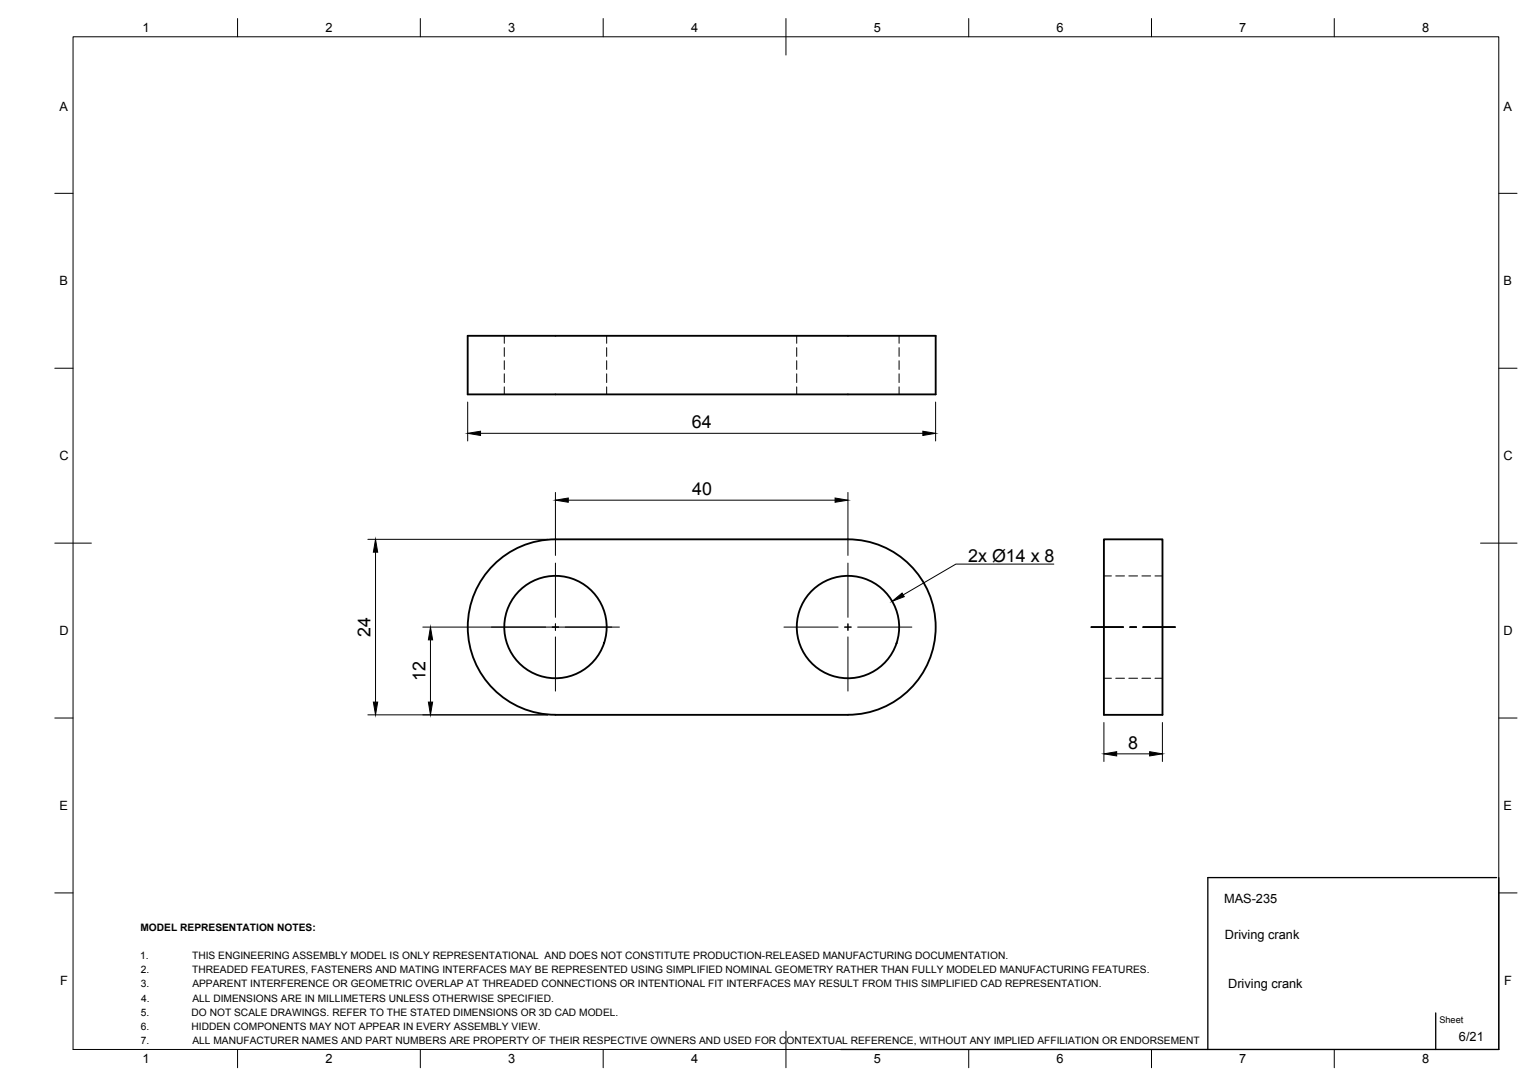
ISO-10303-21;
HEADER;
/* Generated by software containing ST-Developer
 * from STEP Tools, Inc. (www.steptools.com) 
 */

FILE_DESCRIPTION(
/* description */ ('Independent Whitworth quick-return mechanism. Crank radius40, ground-
center spacing80, lever180, connecting rod160, output guide X200. Nomi
nal stroke180 and long/short phase ratio2. Retained guide rods, replac
eable bearing sleeves and captured sliding shoe. No load or production
 rating assigned.'),
/* implementation_level */ '2;1');

FILE_NAME(
/* name */ 'Driving crank.step',
/* time_stamp */ '2026-11-09T18:22:56-08:00',
/* author */ (''),
/* organization */ (''),
/* preprocessor_version */ 'ST-DEVELOPER v20.2',
/* originating_system */ 'Autodesk Translation Framework v15.17.0.0',
/* authorisation */ '');

FILE_SCHEMA (('AUTOMOTIVE_DESIGN { 1 0 10303 214 3 1 1 }'));
ENDSEC;

DATA;
#10=MECHANICAL_DESIGN_GEOMETRIC_PRESENTATION_REPRESENTATION('',(#222),#4388);
#182=SHAPE_REPRESENTATION_RELATIONSHIP('SRR','None',#4481,#202);
#202=ADVANCED_BREP_SHAPE_REPRESENTATION('',(#242),#4371);
#222=STYLED_ITEM('',(#4589),#242);
#242=MANIFOLD_SOLID_BREP('Body1',#2327);
#267=FACE_BOUND('',#583,.T.);
#268=FACE_BOUND('',#584,.T.);
#269=FACE_BOUND('',#586,.T.);
#270=FACE_BOUND('',#587,.T.);
#329=PLANE('',#2604);
#330=PLANE('',#2608);
#331=PLANE('',#2612);
#332=PLANE('',#2613);
#421=FACE_OUTER_BOUND('',#576,.T.);
#422=FACE_OUTER_BOUND('',#577,.T.);
#423=FACE_OUTER_BOUND('',#578,.T.);
#424=FACE_OUTER_BOUND('',#579,.T.);
#425=FACE_OUTER_BOUND('',#580,.T.);
#426=FACE_OUTER_BOUND('',#581,.T.);
#427=FACE_OUTER_BOUND('',#582,.T.);
#428=FACE_OUTER_BOUND('',#585,.T.);
#576=EDGE_LOOP('',(#1654,#1655,#1656,#1657));
#577=EDGE_LOOP('',(#1658,#1659,#1660,#1661));
#578=EDGE_LOOP('',(#1662,#1663,#1664,#1665));
#579=EDGE_LOOP('',(#1666,#1667,#1668,#1669));
#580=EDGE_LOOP('',(#1670,#1671,#1672,#1673));
#581=EDGE_LOOP('',(#1674,#1675,#1676,#1677));
#582=EDGE_LOOP('',(#1678,#1679,#1680,#1681));
#583=EDGE_LOOP('',(#1682));
#584=EDGE_LOOP('',(#1683));
#585=EDGE_LOOP('',(#1684,#1685,#1686,#1687));
#586=EDGE_LOOP('',(#1688));
#587=EDGE_LOOP('',(#1689));
#777=LINE('',#3775,#916);
#778=LINE('',#3781,#917);
#779=LINE('',#3786,#918);
#780=LINE('',#3788,#919);
#781=LINE('',#3790,#920);
#782=LINE('',#3791,#921);
#783=LINE('',#3797,#922);
#784=LINE('',#3800,#923);
#785=LINE('',#3802,#924);
#786=LINE('',#3803,#925);
#916=VECTOR('',#2985,7.);
#917=VECTOR('',#2992,7.);
#918=VECTOR('',#2997,10.);
#919=VECTOR('',#2998,10.);
#920=VECTOR('',#2999,10.);
#921=VECTOR('',#3000,10.);
#922=VECTOR('',#3007,10.);
#923=VECTOR('',#3010,10.);
#924=VECTOR('',#3011,10.);
#925=VECTOR('',#3012,10.);
#1049=CIRCLE('',#2599,7.);
#1050=CIRCLE('',#2600,7.);
#1051=CIRCLE('',#2602,7.);
#1052=CIRCLE('',#2603,7.);
#1053=CIRCLE('',#2606,12.);
#1054=CIRCLE('',#2607,12.);
#1055=CIRCLE('',#2610,12.);
#1056=CIRCLE('',#2611,12.);
#1179=VERTEX_POINT('',#3772);
#1180=VERTEX_POINT('',#3774);
#1181=VERTEX_POINT('',#3778);
#1182=VERTEX_POINT('',#3780);
#1183=VERTEX_POINT('',#3784);
#1184=VERTEX_POINT('',#3785);
#1185=VERTEX_POINT('',#3787);
#1186=VERTEX_POINT('',#3789);
#1187=VERTEX_POINT('',#3793);
#1188=VERTEX_POINT('',#3795);
#1189=VERTEX_POINT('',#3799);
#1190=VERTEX_POINT('',#3801);
#1363=EDGE_CURVE('',#1179,#1179,#1049,.T.);
#1364=EDGE_CURVE('',#1179,#1180,#777,.T.);
#1365=EDGE_CURVE('',#1180,#1180,#1050,.T.);
#1366=EDGE_CURVE('',#1181,#1181,#1051,.T.);
#1367=EDGE_CURVE('',#1181,#1182,#778,.T.);
#1368=EDGE_CURVE('',#1182,#1182,#1052,.T.);
#1369=EDGE_CURVE('',#1183,#1184,#779,.T.);
#1370=EDGE_CURVE('',#1184,#1185,#780,.T.);
#1371=EDGE_CURVE('',#1186,#1185,#781,.T.);
#1372=EDGE_CURVE('',#1183,#1186,#782,.T.);
#1373=EDGE_CURVE('',#1187,#1183,#1053,.T.);
#1374=EDGE_CURVE('',#1188,#1186,#1054,.T.);
#1375=EDGE_CURVE('',#1187,#1188,#783,.T.);
#1376=EDGE_CURVE('',#1189,#1187,#784,.T.);
#1377=EDGE_CURVE('',#1190,#1188,#785,.T.);
#1378=EDGE_CURVE('',#1189,#1190,#786,.T.);
#1379=EDGE_CURVE('',#1184,#1189,#1055,.T.);
#1380=EDGE_CURVE('',#1185,#1190,#1056,.T.);
#1654=ORIENTED_EDGE('',*,*,#1363,.F.);
#1655=ORIENTED_EDGE('',*,*,#1364,.T.);
#1656=ORIENTED_EDGE('',*,*,#1365,.F.);
#1657=ORIENTED_EDGE('',*,*,#1364,.F.);
#1658=ORIENTED_EDGE('',*,*,#1366,.F.);
#1659=ORIENTED_EDGE('',*,*,#1367,.T.);
#1660=ORIENTED_EDGE('',*,*,#1368,.F.);
#1661=ORIENTED_EDGE('',*,*,#1367,.F.);
#1662=ORIENTED_EDGE('',*,*,#1369,.T.);
#1663=ORIENTED_EDGE('',*,*,#1370,.T.);
#1664=ORIENTED_EDGE('',*,*,#1371,.F.);
#1665=ORIENTED_EDGE('',*,*,#1372,.F.);
#1666=ORIENTED_EDGE('',*,*,#1373,.T.);
#1667=ORIENTED_EDGE('',*,*,#1372,.T.);
#1668=ORIENTED_EDGE('',*,*,#1374,.F.);
#1669=ORIENTED_EDGE('',*,*,#1375,.F.);
#1670=ORIENTED_EDGE('',*,*,#1376,.T.);
#1671=ORIENTED_EDGE('',*,*,#1375,.T.);
#1672=ORIENTED_EDGE('',*,*,#1377,.F.);
#1673=ORIENTED_EDGE('',*,*,#1378,.F.);
#1674=ORIENTED_EDGE('',*,*,#1379,.T.);
#1675=ORIENTED_EDGE('',*,*,#1378,.T.);
#1676=ORIENTED_EDGE('',*,*,#1380,.F.);
#1677=ORIENTED_EDGE('',*,*,#1370,.F.);
#1678=ORIENTED_EDGE('',*,*,#1380,.T.);
#1679=ORIENTED_EDGE('',*,*,#1377,.T.);
#1680=ORIENTED_EDGE('',*,*,#1374,.T.);
#1681=ORIENTED_EDGE('',*,*,#1371,.T.);
#1682=ORIENTED_EDGE('',*,*,#1363,.T.);
#1683=ORIENTED_EDGE('',*,*,#1366,.T.);
#1684=ORIENTED_EDGE('',*,*,#1379,.F.);
#1685=ORIENTED_EDGE('',*,*,#1369,.F.);
#1686=ORIENTED_EDGE('',*,*,#1373,.F.);
#1687=ORIENTED_EDGE('',*,*,#1376,.F.);
#1688=ORIENTED_EDGE('',*,*,#1365,.T.);
#1689=ORIENTED_EDGE('',*,*,#1368,.T.);
#2122=CYLINDRICAL_SURFACE('',#2598,7.);
#2123=CYLINDRICAL_SURFACE('',#2601,7.);
#2124=CYLINDRICAL_SURFACE('',#2605,12.);
#2125=CYLINDRICAL_SURFACE('',#2609,12.);
#2193=ADVANCED_FACE('',(#421),#2122,.F.);
#2194=ADVANCED_FACE('',(#422),#2123,.F.);
#2195=ADVANCED_FACE('',(#423),#329,.T.);
#2196=ADVANCED_FACE('',(#424),#2124,.T.);
#2197=ADVANCED_FACE('',(#425),#330,.T.);
#2198=ADVANCED_FACE('',(#426),#2125,.T.);
#2199=ADVANCED_FACE('',(#427,#267,#268),#331,.T.);
#2200=ADVANCED_FACE('',(#428,#269,#270),#332,.F.);
#2327=CLOSED_SHELL('',(#2193,#2194,#2195,#2196,#2197,#2198,#2199,#2200));
#2597=AXIS2_PLACEMENT_3D('',#3770,#2979,#2980);
#2598=AXIS2_PLACEMENT_3D('',#3771,#2981,#2982);
#2599=AXIS2_PLACEMENT_3D('',#3773,#2983,#2984);
#2600=AXIS2_PLACEMENT_3D('',#3776,#2986,#2987);
#2601=AXIS2_PLACEMENT_3D('',#3777,#2988,#2989);
#2602=AXIS2_PLACEMENT_3D('',#3779,#2990,#2991);
#2603=AXIS2_PLACEMENT_3D('',#3782,#2993,#2994);
#2604=AXIS2_PLACEMENT_3D('',#3783,#2995,#2996);
#2605=AXIS2_PLACEMENT_3D('',#3792,#3001,#3002);
#2606=AXIS2_PLACEMENT_3D('',#3794,#3003,#3004);
#2607=AXIS2_PLACEMENT_3D('',#3796,#3005,#3006);
#2608=AXIS2_PLACEMENT_3D('',#3798,#3008,#3009);
#2609=AXIS2_PLACEMENT_3D('',#3804,#3013,#3014);
#2610=AXIS2_PLACEMENT_3D('',#3805,#3015,#3016);
#2611=AXIS2_PLACEMENT_3D('',#3806,#3017,#3018);
#2612=AXIS2_PLACEMENT_3D('',#3807,#3019,#3020);
#2613=AXIS2_PLACEMENT_3D('',#3808,#3021,#3022);
#2979=DIRECTION('axis',(0.,0.,1.));
#2980=DIRECTION('refdir',(1.,0.,0.));
#2981=DIRECTION('center_axis',(0.,0.,-1.));
#2982=DIRECTION('ref_axis',(1.,0.,0.));
#2983=DIRECTION('center_axis',(0.,0.,-1.));
#2984=DIRECTION('ref_axis',(1.,0.,0.));
#2985=DIRECTION('',(0.,0.,-1.));
#2986=DIRECTION('center_axis',(0.,0.,1.));
#2987=DIRECTION('ref_axis',(1.,0.,0.));
#2988=DIRECTION('center_axis',(0.,0.,-1.));
#2989=DIRECTION('ref_axis',(1.,0.,0.));
#2990=DIRECTION('center_axis',(0.,0.,-1.));
#2991=DIRECTION('ref_axis',(1.,0.,0.));
#2992=DIRECTION('',(0.,0.,-1.));
#2993=DIRECTION('center_axis',(0.,0.,1.));
#2994=DIRECTION('ref_axis',(1.,0.,0.));
#2995=DIRECTION('center_axis',(0.,1.,0.));
#2996=DIRECTION('ref_axis',(-1.,0.,0.));
#2997=DIRECTION('',(-1.,0.,0.));
#2998=DIRECTION('',(0.,0.,1.));
#2999=DIRECTION('',(-1.,0.,0.));
#3000=DIRECTION('',(0.,0.,1.));
#3001=DIRECTION('center_axis',(0.,0.,1.));
#3002=DIRECTION('ref_axis',(0.,-1.,0.));
#3003=DIRECTION('center_axis',(0.,0.,1.));
#3004=DIRECTION('ref_axis',(0.,-1.,0.));
#3005=DIRECTION('center_axis',(0.,0.,1.));
#3006=DIRECTION('ref_axis',(0.,-1.,0.));
#3007=DIRECTION('',(0.,0.,1.));
#3008=DIRECTION('center_axis',(0.,-1.,0.));
#3009=DIRECTION('ref_axis',(1.,0.,0.));
#3010=DIRECTION('',(1.,0.,0.));
#3011=DIRECTION('',(1.,0.,0.));
#3012=DIRECTION('',(0.,0.,1.));
#3013=DIRECTION('center_axis',(0.,0.,1.));
#3014=DIRECTION('ref_axis',(0.,1.,0.));
#3015=DIRECTION('center_axis',(0.,0.,1.));
#3016=DIRECTION('ref_axis',(0.,1.,0.));
#3017=DIRECTION('center_axis',(0.,0.,1.));
#3018=DIRECTION('ref_axis',(0.,1.,0.));
#3019=DIRECTION('center_axis',(0.,0.,1.));
#3020=DIRECTION('ref_axis',(1.,0.,0.));
#3021=DIRECTION('center_axis',(0.,0.,1.));
#3022=DIRECTION('ref_axis',(1.,0.,0.));
#3770=CARTESIAN_POINT('',(0.,0.,0.));
#3771=CARTESIAN_POINT('Origin',(0.,0.,4.));
#3772=CARTESIAN_POINT('',(-7.,8.57252759403147E-16,8.));
#3773=CARTESIAN_POINT('Origin',(0.,0.,8.));
#3774=CARTESIAN_POINT('',(-7.,8.57252759403147E-16,0.));
#3775=CARTESIAN_POINT('',(-7.,8.57252759403147E-16,4.));
#3776=CARTESIAN_POINT('Origin',(0.,0.,0.));
#3777=CARTESIAN_POINT('Origin',(40.,0.,4.));
#3778=CARTESIAN_POINT('',(33.,8.57252759403147E-16,8.));
#3779=CARTESIAN_POINT('Origin',(40.,0.,8.));
#3780=CARTESIAN_POINT('',(33.,8.57252759403147E-16,0.));
#3781=CARTESIAN_POINT('',(33.,8.57252759403147E-16,4.));
#3782=CARTESIAN_POINT('Origin',(40.,0.,0.));
#3783=CARTESIAN_POINT('Origin',(40.,12.,0.));
#3784=CARTESIAN_POINT('',(40.,12.,0.));
#3785=CARTESIAN_POINT('',(0.,12.,0.));
#3786=CARTESIAN_POINT('',(40.,12.,0.));
#3787=CARTESIAN_POINT('',(0.,12.,8.));
#3788=CARTESIAN_POINT('',(0.,12.,0.));
#3789=CARTESIAN_POINT('',(40.,12.,8.));
#3790=CARTESIAN_POINT('',(40.,12.,8.));
#3791=CARTESIAN_POINT('',(40.,12.,0.));
#3792=CARTESIAN_POINT('Origin',(40.,0.,0.));
#3793=CARTESIAN_POINT('',(40.,-12.,0.));
#3794=CARTESIAN_POINT('Origin',(40.,0.,0.));
#3795=CARTESIAN_POINT('',(40.,-12.,8.));
#3796=CARTESIAN_POINT('Origin',(40.,0.,8.));
#3797=CARTESIAN_POINT('',(40.,-12.,0.));
#3798=CARTESIAN_POINT('Origin',(0.,-12.,0.));
#3799=CARTESIAN_POINT('',(-1.46957615897682E-15,-12.,0.));
#3800=CARTESIAN_POINT('',(0.,-12.,0.));
#3801=CARTESIAN_POINT('',(-1.46957615897682E-15,-12.,8.));
#3802=CARTESIAN_POINT('',(0.,-12.,8.));
#3803=CARTESIAN_POINT('',(-1.46957615897682E-15,-12.,0.));
#3804=CARTESIAN_POINT('Origin',(0.,0.,0.));
#3805=CARTESIAN_POINT('Origin',(0.,0.,0.));
#3806=CARTESIAN_POINT('Origin',(0.,0.,8.));
#3807=CARTESIAN_POINT('Origin',(20.,0.,8.));
#3808=CARTESIAN_POINT('Origin',(20.,0.,0.));
#4349=UNCERTAINTY_MEASURE_WITH_UNIT(LENGTH_MEASURE(0.01),#4389,
'DISTANCE_ACCURACY_VALUE',
'Maximum model space distance between geometric entities at asserted c
onnectivities');
#4366=UNCERTAINTY_MEASURE_WITH_UNIT(LENGTH_MEASURE(0.01),#4389,
'DISTANCE_ACCURACY_VALUE',
'Maximum model space distance between geometric entities at asserted c
onnectivities');
#4371=(
GEOMETRIC_REPRESENTATION_CONTEXT(3)
GLOBAL_UNCERTAINTY_ASSIGNED_CONTEXT((#4349))
GLOBAL_UNIT_ASSIGNED_CONTEXT((#4389,#4391,#4392))
REPRESENTATION_CONTEXT('','3D')
);
#4388=(
GEOMETRIC_REPRESENTATION_CONTEXT(3)
GLOBAL_UNCERTAINTY_ASSIGNED_CONTEXT((#4366))
GLOBAL_UNIT_ASSIGNED_CONTEXT((#4389,#4391,#4392))
REPRESENTATION_CONTEXT('','3D')
);
#4389=(
LENGTH_UNIT()
NAMED_UNIT(*)
SI_UNIT(.MILLI.,.METRE.)
);
#4391=(
NAMED_UNIT(*)
PLANE_ANGLE_UNIT()
SI_UNIT($,.RADIAN.)
);
#4392=(
NAMED_UNIT(*)
SI_UNIT($,.STERADIAN.)
SOLID_ANGLE_UNIT()
);
#4397=SHAPE_DEFINITION_REPRESENTATION(#4418,#4481);
#4418=PRODUCT_DEFINITION_SHAPE('',$,#4503);
#4481=SHAPE_REPRESENTATION('',(#2597),#4371);
#4498=PRODUCT_DEFINITION_CONTEXT('part definition',#4563,'design');
#4503=PRODUCT_DEFINITION('Driving crank','Driving crank',#4524,#4498);
#4524=PRODUCT_DEFINITION_FORMATION('',$,#4569);
#4563=APPLICATION_CONTEXT(
'Core Data for Automotive Mechanical Design Process');
#4564=PRODUCT_CONTEXT('part definition',#4563,'mechanical');
#4569=PRODUCT('Driving crank','Driving crank','Driving crank',(#4564));
#4589=PRESENTATION_STYLE_ASSIGNMENT((#4603));
#4603=SURFACE_STYLE_USAGE(.BOTH.,#4617);
#4617=SURFACE_SIDE_STYLE('',(#4631));
#4631=SURFACE_STYLE_FILL_AREA(#4645);
#4645=FILL_AREA_STYLE('Driving crank finish',(#4659));
#4659=FILL_AREA_STYLE_COLOUR('Driving crank finish',#4673);
#4673=COLOUR_RGB('Driving crank finish',0.0901960784313725,0.270588235294118,
0.513725490196078);
ENDSEC;
END-ISO-10303-21;
